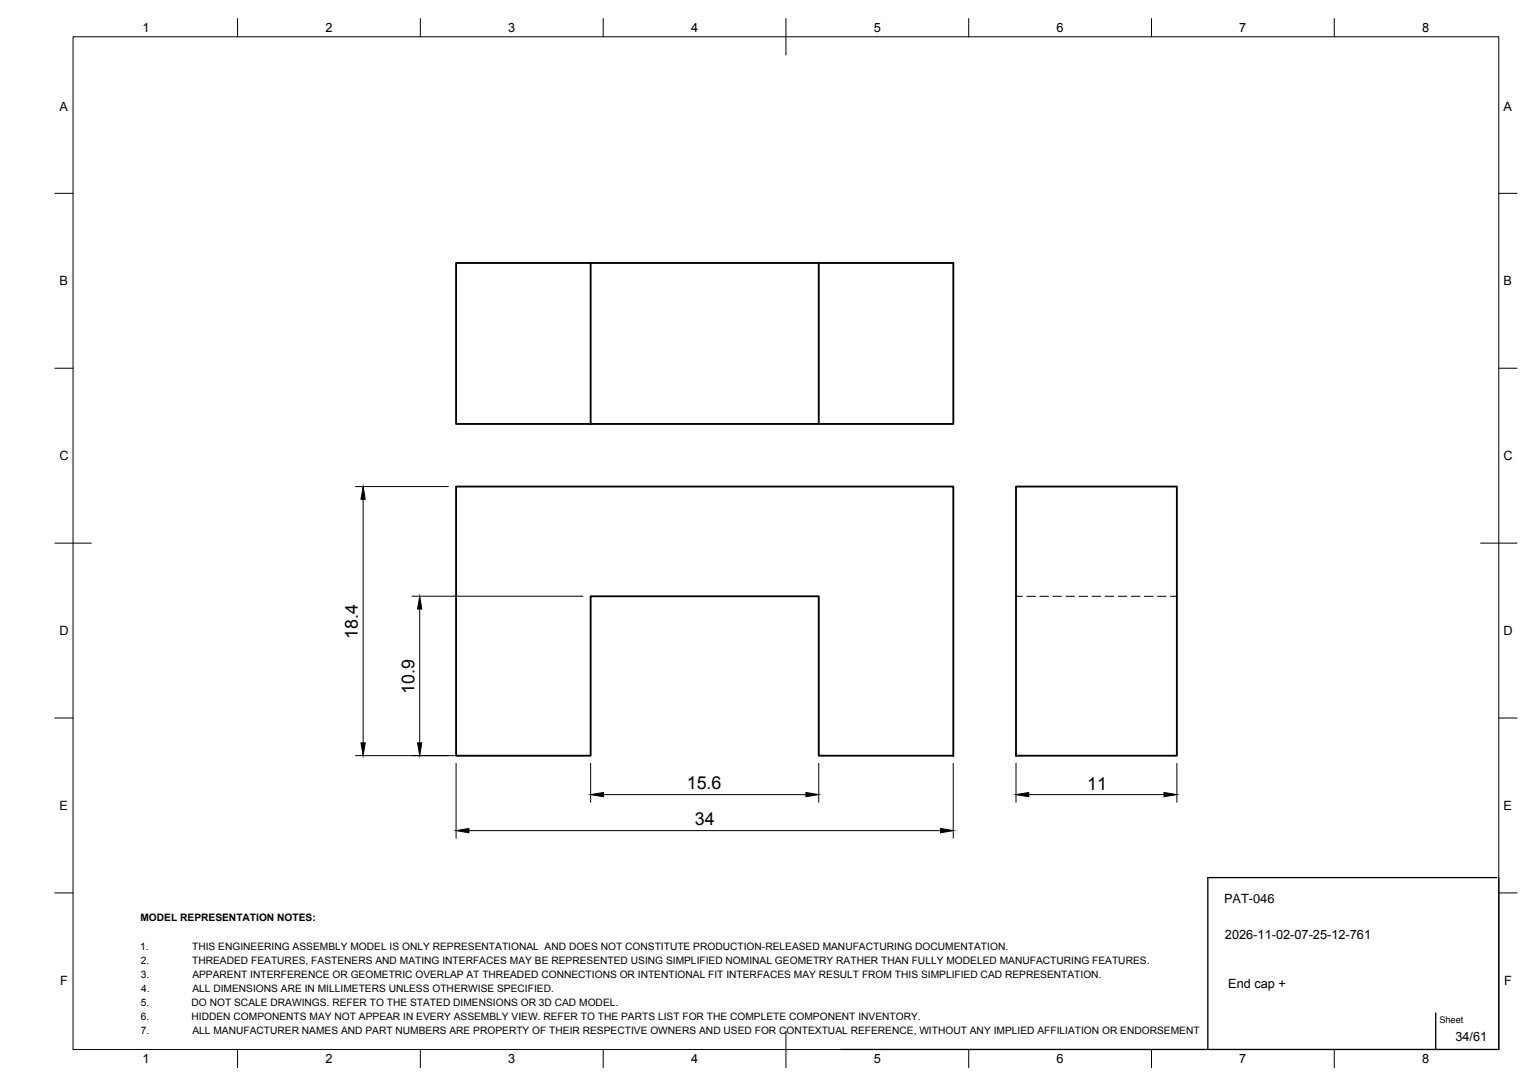
ISO-10303-21;
HEADER;
/* Generated by software containing ST-Developer
 * from STEP Tools, Inc. (www.steptools.com) 
 */

FILE_DESCRIPTION(
/* description */ ('Gear mesh backlash fixture'),
/* implementation_level */ '2;1');

FILE_NAME(
/* name */ 'End cap +.step',
/* time_stamp */ '2026-10-28T03:26:00-07:00',
/* author */ (''),
/* organization */ (''),
/* preprocessor_version */ 'ST-DEVELOPER v20.2',
/* originating_system */ 'Autodesk Translation Framework v15.17.0.0',
/* authorisation */ '');

FILE_SCHEMA (('AUTOMOTIVE_DESIGN { 1 0 10303 214 3 1 1 }'));
ENDSEC;

DATA;
#10=MECHANICAL_DESIGN_GEOMETRIC_PRESENTATION_REPRESENTATION('',(#1047),#57900);
#940=SHAPE_REPRESENTATION_RELATIONSHIP('SRR','None',#58138,#990);
#990=ADVANCED_BREP_SHAPE_REPRESENTATION('',(#1111),#57871);
#1047=STYLED_ITEM('',(#58458),#1111);
#1111=MANIFOLD_SOLID_BREP('Body1',#13608);
#1492=PLANE('',#14842);
#1493=PLANE('',#14843);
#1494=PLANE('',#14844);
#1495=PLANE('',#14845);
#1496=PLANE('',#14846);
#1497=PLANE('',#14847);
#1498=PLANE('',#14848);
#1499=PLANE('',#14849);
#1500=PLANE('',#14850);
#1501=PLANE('',#14851);
#1996=FACE_OUTER_BOUND('',#2898,.T.);
#1997=FACE_OUTER_BOUND('',#2899,.T.);
#1998=FACE_OUTER_BOUND('',#2900,.T.);
#1999=FACE_OUTER_BOUND('',#2901,.T.);
#2000=FACE_OUTER_BOUND('',#2902,.T.);
#2001=FACE_OUTER_BOUND('',#2903,.T.);
#2002=FACE_OUTER_BOUND('',#2904,.T.);
#2003=FACE_OUTER_BOUND('',#2905,.T.);
#2004=FACE_OUTER_BOUND('',#2906,.T.);
#2005=FACE_OUTER_BOUND('',#2907,.T.);
#2898=EDGE_LOOP('',(#10269,#10270,#10271,#10272));
#2899=EDGE_LOOP('',(#10273,#10274,#10275,#10276));
#2900=EDGE_LOOP('',(#10277,#10278,#10279,#10280));
#2901=EDGE_LOOP('',(#10281,#10282,#10283,#10284));
#2902=EDGE_LOOP('',(#10285,#10286,#10287,#10288));
#2903=EDGE_LOOP('',(#10289,#10290,#10291,#10292));
#2904=EDGE_LOOP('',(#10293,#10294,#10295,#10296));
#2905=EDGE_LOOP('',(#10297,#10298,#10299,#10300));
#2906=EDGE_LOOP('',(#10301,#10302,#10303,#10304,#10305,#10306,#10307,#10308));
#2907=EDGE_LOOP('',(#10309,#10310,#10311,#10312,#10313,#10314,#10315,#10316));
#3771=LINE('',#21191,#4660);
#3772=LINE('',#21193,#4661);
#3773=LINE('',#21195,#4662);
#3774=LINE('',#21196,#4663);
#3775=LINE('',#21199,#4664);
#3776=LINE('',#21201,#4665);
#3777=LINE('',#21202,#4666);
#3778=LINE('',#21205,#4667);
#3779=LINE('',#21207,#4668);
#3780=LINE('',#21208,#4669);
#3781=LINE('',#21211,#4670);
#3782=LINE('',#21213,#4671);
#3783=LINE('',#21214,#4672);
#3784=LINE('',#21217,#4673);
#3785=LINE('',#21219,#4674);
#3786=LINE('',#21220,#4675);
#3787=LINE('',#21223,#4676);
#3788=LINE('',#21225,#4677);
#3789=LINE('',#21226,#4678);
#3790=LINE('',#21229,#4679);
#3791=LINE('',#21231,#4680);
#3792=LINE('',#21232,#4681);
#3793=LINE('',#21234,#4682);
#3794=LINE('',#21235,#4683);
#4660=VECTOR('',#17234,1.);
#4661=VECTOR('',#17235,1.);
#4662=VECTOR('',#17236,1.);
#4663=VECTOR('',#17237,1.);
#4664=VECTOR('',#17240,1.);
#4665=VECTOR('',#17241,1.);
#4666=VECTOR('',#17242,1.);
#4667=VECTOR('',#17245,1.);
#4668=VECTOR('',#17246,1.);
#4669=VECTOR('',#17247,1.);
#4670=VECTOR('',#17250,1.);
#4671=VECTOR('',#17251,1.);
#4672=VECTOR('',#17252,1.);
#4673=VECTOR('',#17255,1.);
#4674=VECTOR('',#17256,1.);
#4675=VECTOR('',#17257,1.);
#4676=VECTOR('',#17260,1.);
#4677=VECTOR('',#17261,1.);
#4678=VECTOR('',#17262,1.);
#4679=VECTOR('',#17265,1.);
#4680=VECTOR('',#17266,1.);
#4681=VECTOR('',#17267,1.);
#4682=VECTOR('',#17270,1.);
#4683=VECTOR('',#17271,1.);
#6247=VERTEX_POINT('',#21189);
#6248=VERTEX_POINT('',#21190);
#6249=VERTEX_POINT('',#21192);
#6250=VERTEX_POINT('',#21194);
#6251=VERTEX_POINT('',#21198);
#6252=VERTEX_POINT('',#21200);
#6253=VERTEX_POINT('',#21204);
#6254=VERTEX_POINT('',#21206);
#6255=VERTEX_POINT('',#21210);
#6256=VERTEX_POINT('',#21212);
#6257=VERTEX_POINT('',#21216);
#6258=VERTEX_POINT('',#21218);
#6259=VERTEX_POINT('',#21222);
#6260=VERTEX_POINT('',#21224);
#6261=VERTEX_POINT('',#21228);
#6262=VERTEX_POINT('',#21230);
#7721=EDGE_CURVE('',#6247,#6248,#3771,.T.);
#7722=EDGE_CURVE('',#6248,#6249,#3772,.T.);
#7723=EDGE_CURVE('',#6250,#6249,#3773,.T.);
#7724=EDGE_CURVE('',#6247,#6250,#3774,.T.);
#7725=EDGE_CURVE('',#6251,#6247,#3775,.T.);
#7726=EDGE_CURVE('',#6252,#6250,#3776,.T.);
#7727=EDGE_CURVE('',#6251,#6252,#3777,.T.);
#7728=EDGE_CURVE('',#6253,#6251,#3778,.T.);
#7729=EDGE_CURVE('',#6254,#6252,#3779,.T.);
#7730=EDGE_CURVE('',#6253,#6254,#3780,.T.);
#7731=EDGE_CURVE('',#6255,#6253,#3781,.T.);
#7732=EDGE_CURVE('',#6256,#6254,#3782,.T.);
#7733=EDGE_CURVE('',#6255,#6256,#3783,.T.);
#7734=EDGE_CURVE('',#6257,#6255,#3784,.T.);
#7735=EDGE_CURVE('',#6258,#6256,#3785,.T.);
#7736=EDGE_CURVE('',#6257,#6258,#3786,.T.);
#7737=EDGE_CURVE('',#6259,#6257,#3787,.T.);
#7738=EDGE_CURVE('',#6260,#6258,#3788,.T.);
#7739=EDGE_CURVE('',#6259,#6260,#3789,.T.);
#7740=EDGE_CURVE('',#6261,#6259,#3790,.T.);
#7741=EDGE_CURVE('',#6262,#6260,#3791,.T.);
#7742=EDGE_CURVE('',#6261,#6262,#3792,.T.);
#7743=EDGE_CURVE('',#6248,#6261,#3793,.T.);
#7744=EDGE_CURVE('',#6249,#6262,#3794,.T.);
#10269=ORIENTED_EDGE('',*,*,#7721,.T.);
#10270=ORIENTED_EDGE('',*,*,#7722,.T.);
#10271=ORIENTED_EDGE('',*,*,#7723,.F.);
#10272=ORIENTED_EDGE('',*,*,#7724,.F.);
#10273=ORIENTED_EDGE('',*,*,#7725,.T.);
#10274=ORIENTED_EDGE('',*,*,#7724,.T.);
#10275=ORIENTED_EDGE('',*,*,#7726,.F.);
#10276=ORIENTED_EDGE('',*,*,#7727,.F.);
#10277=ORIENTED_EDGE('',*,*,#7728,.T.);
#10278=ORIENTED_EDGE('',*,*,#7727,.T.);
#10279=ORIENTED_EDGE('',*,*,#7729,.F.);
#10280=ORIENTED_EDGE('',*,*,#7730,.F.);
#10281=ORIENTED_EDGE('',*,*,#7731,.T.);
#10282=ORIENTED_EDGE('',*,*,#7730,.T.);
#10283=ORIENTED_EDGE('',*,*,#7732,.F.);
#10284=ORIENTED_EDGE('',*,*,#7733,.F.);
#10285=ORIENTED_EDGE('',*,*,#7734,.T.);
#10286=ORIENTED_EDGE('',*,*,#7733,.T.);
#10287=ORIENTED_EDGE('',*,*,#7735,.F.);
#10288=ORIENTED_EDGE('',*,*,#7736,.F.);
#10289=ORIENTED_EDGE('',*,*,#7737,.T.);
#10290=ORIENTED_EDGE('',*,*,#7736,.T.);
#10291=ORIENTED_EDGE('',*,*,#7738,.F.);
#10292=ORIENTED_EDGE('',*,*,#7739,.F.);
#10293=ORIENTED_EDGE('',*,*,#7740,.T.);
#10294=ORIENTED_EDGE('',*,*,#7739,.T.);
#10295=ORIENTED_EDGE('',*,*,#7741,.F.);
#10296=ORIENTED_EDGE('',*,*,#7742,.F.);
#10297=ORIENTED_EDGE('',*,*,#7743,.T.);
#10298=ORIENTED_EDGE('',*,*,#7742,.T.);
#10299=ORIENTED_EDGE('',*,*,#7744,.F.);
#10300=ORIENTED_EDGE('',*,*,#7722,.F.);
#10301=ORIENTED_EDGE('',*,*,#7744,.T.);
#10302=ORIENTED_EDGE('',*,*,#7741,.T.);
#10303=ORIENTED_EDGE('',*,*,#7738,.T.);
#10304=ORIENTED_EDGE('',*,*,#7735,.T.);
#10305=ORIENTED_EDGE('',*,*,#7732,.T.);
#10306=ORIENTED_EDGE('',*,*,#7729,.T.);
#10307=ORIENTED_EDGE('',*,*,#7726,.T.);
#10308=ORIENTED_EDGE('',*,*,#7723,.T.);
#10309=ORIENTED_EDGE('',*,*,#7743,.F.);
#10310=ORIENTED_EDGE('',*,*,#7721,.F.);
#10311=ORIENTED_EDGE('',*,*,#7725,.F.);
#10312=ORIENTED_EDGE('',*,*,#7728,.F.);
#10313=ORIENTED_EDGE('',*,*,#7731,.F.);
#10314=ORIENTED_EDGE('',*,*,#7734,.F.);
#10315=ORIENTED_EDGE('',*,*,#7737,.F.);
#10316=ORIENTED_EDGE('',*,*,#7740,.F.);
#13113=ADVANCED_FACE('',(#1996),#1492,.T.);
#13114=ADVANCED_FACE('',(#1997),#1493,.T.);
#13115=ADVANCED_FACE('',(#1998),#1494,.T.);
#13116=ADVANCED_FACE('',(#1999),#1495,.T.);
#13117=ADVANCED_FACE('',(#2000),#1496,.T.);
#13118=ADVANCED_FACE('',(#2001),#1497,.T.);
#13119=ADVANCED_FACE('',(#2002),#1498,.T.);
#13120=ADVANCED_FACE('',(#2003),#1499,.T.);
#13121=ADVANCED_FACE('',(#2004),#1500,.T.);
#13122=ADVANCED_FACE('',(#2005),#1501,.F.);
#13608=CLOSED_SHELL('',(#13113,#13114,#13115,#13116,#13117,#13118,#13119,
#13120,#13121,#13122));
#14841=AXIS2_PLACEMENT_3D('',#21187,#17230,#17231);
#14842=AXIS2_PLACEMENT_3D('',#21188,#17232,#17233);
#14843=AXIS2_PLACEMENT_3D('',#21197,#17238,#17239);
#14844=AXIS2_PLACEMENT_3D('',#21203,#17243,#17244);
#14845=AXIS2_PLACEMENT_3D('',#21209,#17248,#17249);
#14846=AXIS2_PLACEMENT_3D('',#21215,#17253,#17254);
#14847=AXIS2_PLACEMENT_3D('',#21221,#17258,#17259);
#14848=AXIS2_PLACEMENT_3D('',#21227,#17263,#17264);
#14849=AXIS2_PLACEMENT_3D('',#21233,#17268,#17269);
#14850=AXIS2_PLACEMENT_3D('',#21236,#17272,#17273);
#14851=AXIS2_PLACEMENT_3D('',#21237,#17274,#17275);
#17230=DIRECTION('axis',(0.,0.,1.));
#17231=DIRECTION('refdir',(1.,0.,0.));
#17232=DIRECTION('center_axis',(0.,0.,1.));
#17233=DIRECTION('ref_axis',(0.,-1.,0.));
#17234=DIRECTION('',(0.,-1.,0.));
#17235=DIRECTION('',(1.,0.,0.));
#17236=DIRECTION('',(0.,-1.,0.));
#17237=DIRECTION('',(1.,0.,0.));
#17238=DIRECTION('center_axis',(0.,1.,0.));
#17239=DIRECTION('ref_axis',(0.,0.,1.));
#17240=DIRECTION('',(0.,0.,1.));
#17241=DIRECTION('',(0.,0.,1.));
#17242=DIRECTION('',(1.,0.,0.));
#17243=DIRECTION('center_axis',(0.,0.,-1.));
#17244=DIRECTION('ref_axis',(0.,1.,0.));
#17245=DIRECTION('',(0.,1.,0.));
#17246=DIRECTION('',(0.,1.,0.));
#17247=DIRECTION('',(1.,0.,0.));
#17248=DIRECTION('center_axis',(0.,-1.,0.));
#17249=DIRECTION('ref_axis',(0.,0.,-1.));
#17250=DIRECTION('',(0.,0.,-1.));
#17251=DIRECTION('',(0.,0.,-1.));
#17252=DIRECTION('',(1.,0.,0.));
#17253=DIRECTION('center_axis',(0.,0.,-1.));
#17254=DIRECTION('ref_axis',(0.,1.,0.));
#17255=DIRECTION('',(0.,1.,0.));
#17256=DIRECTION('',(0.,1.,0.));
#17257=DIRECTION('',(1.,0.,0.));
#17258=DIRECTION('center_axis',(0.,1.,0.));
#17259=DIRECTION('ref_axis',(0.,0.,1.));
#17260=DIRECTION('',(0.,0.,1.));
#17261=DIRECTION('',(0.,0.,1.));
#17262=DIRECTION('',(1.,0.,0.));
#17263=DIRECTION('center_axis',(0.,0.,-1.));
#17264=DIRECTION('ref_axis',(0.,1.,0.));
#17265=DIRECTION('',(0.,1.,0.));
#17266=DIRECTION('',(0.,1.,0.));
#17267=DIRECTION('',(1.,0.,0.));
#17268=DIRECTION('center_axis',(0.,-1.,0.));
#17269=DIRECTION('ref_axis',(0.,0.,-1.));
#17270=DIRECTION('',(0.,0.,-1.));
#17271=DIRECTION('',(0.,0.,-1.));
#17272=DIRECTION('center_axis',(1.,0.,0.));
#17273=DIRECTION('ref_axis',(0.,0.,-1.));
#17274=DIRECTION('center_axis',(1.,0.,0.));
#17275=DIRECTION('ref_axis',(0.,0.,-1.));
#21187=CARTESIAN_POINT('',(0.,0.,0.));
#21188=CARTESIAN_POINT('Origin',(1.97,1.7,2.3));
#21189=CARTESIAN_POINT('',(1.97,1.7,2.3));
#21190=CARTESIAN_POINT('',(1.97,-1.7,2.3));
#21191=CARTESIAN_POINT('',(1.97,1.7,2.3));
#21192=CARTESIAN_POINT('',(3.07,-1.7,2.3));
#21193=CARTESIAN_POINT('',(1.97,-1.7,2.3));
#21194=CARTESIAN_POINT('',(3.07,1.7,2.3));
#21195=CARTESIAN_POINT('',(3.07,1.7,2.3));
#21196=CARTESIAN_POINT('',(1.97,1.7,2.3));
#21197=CARTESIAN_POINT('Origin',(1.97,1.7,0.46));
#21198=CARTESIAN_POINT('',(1.97,1.7,0.46));
#21199=CARTESIAN_POINT('',(1.97,1.7,0.46));
#21200=CARTESIAN_POINT('',(3.07,1.7,0.46));
#21201=CARTESIAN_POINT('',(3.07,1.7,0.46));
#21202=CARTESIAN_POINT('',(1.97,1.7,0.46));
#21203=CARTESIAN_POINT('Origin',(1.97,0.78,0.46));
#21204=CARTESIAN_POINT('',(1.97,0.78,0.46));
#21205=CARTESIAN_POINT('',(1.97,0.78,0.46));
#21206=CARTESIAN_POINT('',(3.07,0.78,0.46));
#21207=CARTESIAN_POINT('',(3.07,0.78,0.46));
#21208=CARTESIAN_POINT('',(1.97,0.78,0.46));
#21209=CARTESIAN_POINT('Origin',(1.97,0.78,1.55));
#21210=CARTESIAN_POINT('',(1.97,0.78,1.55));
#21211=CARTESIAN_POINT('',(1.97,0.78,1.55));
#21212=CARTESIAN_POINT('',(3.07,0.78,1.55));
#21213=CARTESIAN_POINT('',(3.07,0.78,1.55));
#21214=CARTESIAN_POINT('',(1.97,0.78,1.55));
#21215=CARTESIAN_POINT('Origin',(1.97,-0.78,1.55));
#21216=CARTESIAN_POINT('',(1.97,-0.78,1.55));
#21217=CARTESIAN_POINT('',(1.97,-0.78,1.55));
#21218=CARTESIAN_POINT('',(3.07,-0.78,1.55));
#21219=CARTESIAN_POINT('',(3.07,-0.78,1.55));
#21220=CARTESIAN_POINT('',(1.97,-0.78,1.55));
#21221=CARTESIAN_POINT('Origin',(1.97,-0.78,0.46));
#21222=CARTESIAN_POINT('',(1.97,-0.78,0.46));
#21223=CARTESIAN_POINT('',(1.97,-0.78,0.46));
#21224=CARTESIAN_POINT('',(3.07,-0.78,0.46));
#21225=CARTESIAN_POINT('',(3.07,-0.78,0.46));
#21226=CARTESIAN_POINT('',(1.97,-0.78,0.46));
#21227=CARTESIAN_POINT('Origin',(1.97,-1.7,0.46));
#21228=CARTESIAN_POINT('',(1.97,-1.7,0.46));
#21229=CARTESIAN_POINT('',(1.97,-1.7,0.46));
#21230=CARTESIAN_POINT('',(3.07,-1.7,0.46));
#21231=CARTESIAN_POINT('',(3.07,-1.7,0.46));
#21232=CARTESIAN_POINT('',(1.97,-1.7,0.46));
#21233=CARTESIAN_POINT('Origin',(1.97,-1.7,2.3));
#21234=CARTESIAN_POINT('',(1.97,-1.7,2.3));
#21235=CARTESIAN_POINT('',(3.07,-1.7,2.3));
#21236=CARTESIAN_POINT('Origin',(3.07,0.,1.38));
#21237=CARTESIAN_POINT('Origin',(1.97,0.,1.38));
#57812=UNCERTAINTY_MEASURE_WITH_UNIT(LENGTH_MEASURE(0.001),#57901,
'DISTANCE_ACCURACY_VALUE',
'Maximum model space distance between geometric entities at asserted c
onnectivities');
#57841=UNCERTAINTY_MEASURE_WITH_UNIT(LENGTH_MEASURE(0.001),#57901,
'DISTANCE_ACCURACY_VALUE',
'Maximum model space distance between geometric entities at asserted c
onnectivities');
#57871=(
GEOMETRIC_REPRESENTATION_CONTEXT(3)
GLOBAL_UNCERTAINTY_ASSIGNED_CONTEXT((#57812))
GLOBAL_UNIT_ASSIGNED_CONTEXT((#57901,#57903,#57904))
REPRESENTATION_CONTEXT('','3D')
);
#57900=(
GEOMETRIC_REPRESENTATION_CONTEXT(3)
GLOBAL_UNCERTAINTY_ASSIGNED_CONTEXT((#57841))
GLOBAL_UNIT_ASSIGNED_CONTEXT((#57901,#57903,#57904))
REPRESENTATION_CONTEXT('','3D')
);
#57901=(
LENGTH_UNIT()
NAMED_UNIT(*)
SI_UNIT(.CENTI.,.METRE.)
);
#57903=(
NAMED_UNIT(*)
PLANE_ANGLE_UNIT()
SI_UNIT($,.RADIAN.)
);
#57904=(
NAMED_UNIT(*)
SI_UNIT($,.STERADIAN.)
SOLID_ANGLE_UNIT()
);
#57934=SHAPE_DEFINITION_REPRESENTATION(#57997,#58138);
#57997=PRODUCT_DEFINITION_SHAPE('',$,#58197);
#58138=SHAPE_REPRESENTATION('',(#14841),#57871);
#58167=PRODUCT_DEFINITION_CONTEXT('part definition',#58343,'design');
#58197=PRODUCT_DEFINITION('End cap +','End cap +',#58255,#58167);
#58255=PRODUCT_DEFINITION_FORMATION('',$,#58374);
#58343=APPLICATION_CONTEXT(
'Core Data for Automotive Mechanical Design Process');
#58344=PRODUCT_CONTEXT('part definition',#58343,'mechanical');
#58374=PRODUCT('End cap +','End cap +','End cap +',(#58344));
#58452=COLOUR_RGB('Sky Blue',0.24,0.69,0.87);
#58453=FILL_AREA_STYLE_COLOUR('',#58452);
#58454=FILL_AREA_STYLE('',(#58453));
#58455=SURFACE_STYLE_FILL_AREA(#58454);
#58456=SURFACE_SIDE_STYLE('',(#58455));
#58457=SURFACE_STYLE_USAGE(.BOTH.,#58456);
#58458=PRESENTATION_STYLE_ASSIGNMENT((#58457));
ENDSEC;
END-ISO-10303-21;
